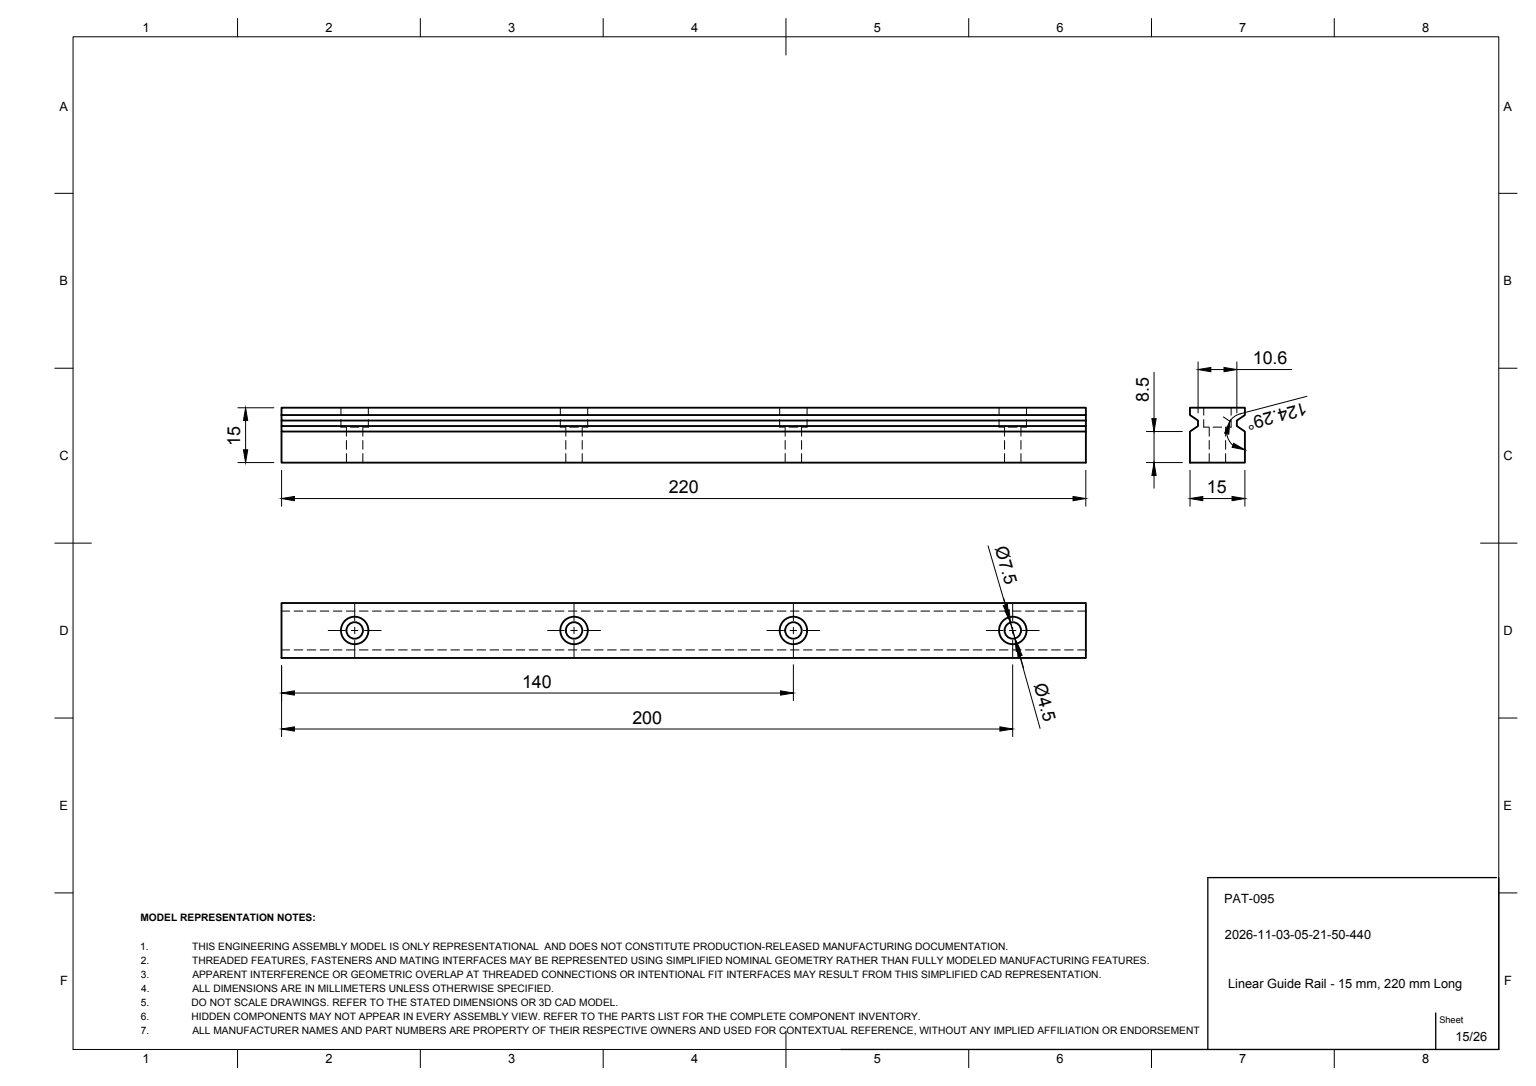
ISO-10303-21;
HEADER;
/* Generated by software containing ST-Developer
 * from STEP Tools, Inc. (www.steptools.com) 
 */

FILE_DESCRIPTION(
/* description */ ('Single-Axis Profile-Rail Linear Slide'),
/* implementation_level */ '2;1');

FILE_NAME(
/* name */ 'Linear Guide Rail - 15 mm, 220 mm Long.step',
/* time_stamp */ '2026-10-27T10:47:43-07:00',
/* author */ (''),
/* organization */ (''),
/* preprocessor_version */ 'ST-DEVELOPER v20.2',
/* originating_system */ 'Autodesk Translation Framework v15.17.0.0',
/* authorisation */ '');

FILE_SCHEMA (('AUTOMOTIVE_DESIGN { 1 0 10303 214 3 1 1 }'));
ENDSEC;

DATA;
#10=MECHANICAL_DESIGN_GEOMETRIC_PRESENTATION_REPRESENTATION('',(#339),#14478);
#285=SHAPE_REPRESENTATION_RELATIONSHIP('SRR','None',#14615,#312);
#312=ADVANCED_BREP_SHAPE_REPRESENTATION('',(#366),#14459);
#339=STYLED_ITEM('',(#14824),#366);
#366=MANIFOLD_SOLID_BREP('Body1',#8599);
#422=FACE_BOUND('',#1545,.T.);
#423=FACE_BOUND('',#1548,.T.);
#424=FACE_BOUND('',#1551,.T.);
#425=FACE_BOUND('',#1554,.T.);
#426=FACE_BOUND('',#1564,.T.);
#427=FACE_BOUND('',#1565,.T.);
#428=FACE_BOUND('',#1566,.T.);
#429=FACE_BOUND('',#1567,.T.);
#430=FACE_BOUND('',#1574,.T.);
#431=FACE_BOUND('',#1575,.T.);
#432=FACE_BOUND('',#1576,.T.);
#433=FACE_BOUND('',#1577,.T.);
#648=PLANE('',#9187);
#649=PLANE('',#9192);
#650=PLANE('',#9197);
#651=PLANE('',#9202);
#652=PLANE('',#9212);
#653=PLANE('',#9213);
#654=PLANE('',#9214);
#655=PLANE('',#9215);
#656=PLANE('',#9216);
#657=PLANE('',#9217);
#658=PLANE('',#9218);
#659=PLANE('',#9219);
#660=PLANE('',#9220);
#661=PLANE('',#9221);
#662=PLANE('',#9222);
#663=PLANE('',#9223);
#664=PLANE('',#9224);
#665=PLANE('',#9225);
#1044=FACE_OUTER_BOUND('',#1543,.T.);
#1045=FACE_OUTER_BOUND('',#1544,.T.);
#1046=FACE_OUTER_BOUND('',#1546,.T.);
#1047=FACE_OUTER_BOUND('',#1547,.T.);
#1048=FACE_OUTER_BOUND('',#1549,.T.);
#1049=FACE_OUTER_BOUND('',#1550,.T.);
#1050=FACE_OUTER_BOUND('',#1552,.T.);
#1051=FACE_OUTER_BOUND('',#1553,.T.);
#1052=FACE_OUTER_BOUND('',#1555,.T.);
#1053=FACE_OUTER_BOUND('',#1556,.T.);
#1054=FACE_OUTER_BOUND('',#1557,.T.);
#1055=FACE_OUTER_BOUND('',#1558,.T.);
#1056=FACE_OUTER_BOUND('',#1559,.T.);
#1057=FACE_OUTER_BOUND('',#1560,.T.);
#1058=FACE_OUTER_BOUND('',#1561,.T.);
#1059=FACE_OUTER_BOUND('',#1562,.T.);
#1060=FACE_OUTER_BOUND('',#1563,.T.);
#1061=FACE_OUTER_BOUND('',#1568,.T.);
#1062=FACE_OUTER_BOUND('',#1569,.T.);
#1063=FACE_OUTER_BOUND('',#1570,.T.);
#1064=FACE_OUTER_BOUND('',#1571,.T.);
#1065=FACE_OUTER_BOUND('',#1572,.T.);
#1066=FACE_OUTER_BOUND('',#1573,.T.);
#1067=FACE_OUTER_BOUND('',#1578,.T.);
#1068=FACE_OUTER_BOUND('',#1579,.T.);
#1069=FACE_OUTER_BOUND('',#1580,.T.);
#1543=EDGE_LOOP('',(#6893,#6894,#6895,#6896));
#1544=EDGE_LOOP('',(#6897));
#1545=EDGE_LOOP('',(#6898));
#1546=EDGE_LOOP('',(#6899,#6900,#6901,#6902));
#1547=EDGE_LOOP('',(#6903));
#1548=EDGE_LOOP('',(#6904));
#1549=EDGE_LOOP('',(#6905,#6906,#6907,#6908));
#1550=EDGE_LOOP('',(#6909));
#1551=EDGE_LOOP('',(#6910));
#1552=EDGE_LOOP('',(#6911,#6912,#6913,#6914));
#1553=EDGE_LOOP('',(#6915));
#1554=EDGE_LOOP('',(#6916));
#1555=EDGE_LOOP('',(#6917,#6918,#6919,#6920));
#1556=EDGE_LOOP('',(#6921,#6922,#6923,#6924));
#1557=EDGE_LOOP('',(#6925,#6926,#6927,#6928));
#1558=EDGE_LOOP('',(#6929,#6930,#6931,#6932));
#1559=EDGE_LOOP('',(#6933,#6934,#6935,#6936));
#1560=EDGE_LOOP('',(#6937,#6938,#6939,#6940));
#1561=EDGE_LOOP('',(#6941,#6942,#6943,#6944));
#1562=EDGE_LOOP('',(#6945,#6946,#6947,#6948));
#1563=EDGE_LOOP('',(#6949,#6950,#6951,#6952));
#1564=EDGE_LOOP('',(#6953));
#1565=EDGE_LOOP('',(#6954));
#1566=EDGE_LOOP('',(#6955));
#1567=EDGE_LOOP('',(#6956));
#1568=EDGE_LOOP('',(#6957,#6958,#6959,#6960));
#1569=EDGE_LOOP('',(#6961,#6962,#6963,#6964));
#1570=EDGE_LOOP('',(#6965,#6966,#6967,#6968));
#1571=EDGE_LOOP('',(#6969,#6970,#6971,#6972));
#1572=EDGE_LOOP('',(#6973,#6974,#6975,#6976));
#1573=EDGE_LOOP('',(#6977,#6978,#6979,#6980));
#1574=EDGE_LOOP('',(#6981));
#1575=EDGE_LOOP('',(#6982));
#1576=EDGE_LOOP('',(#6983));
#1577=EDGE_LOOP('',(#6984));
#1578=EDGE_LOOP('',(#6985,#6986,#6987,#6988));
#1579=EDGE_LOOP('',(#6989,#6990,#6991,#6992,#6993,#6994,#6995,#6996,#6997,
#6998,#6999,#7000));
#1580=EDGE_LOOP('',(#7001,#7002,#7003,#7004,#7005,#7006,#7007,#7008,#7009,
#7010,#7011,#7012));
#2332=LINE('',#13117,#3303);
#2333=LINE('',#13126,#3304);
#2334=LINE('',#13135,#3305);
#2335=LINE('',#13144,#3306);
#2336=LINE('',#13152,#3307);
#2337=LINE('',#13156,#3308);
#2338=LINE('',#13160,#3309);
#2339=LINE('',#13164,#3310);
#2340=LINE('',#13168,#3311);
#2341=LINE('',#13170,#3312);
#2342=LINE('',#13172,#3313);
#2343=LINE('',#13173,#3314);
#2344=LINE('',#13176,#3315);
#2345=LINE('',#13178,#3316);
#2346=LINE('',#13179,#3317);
#2347=LINE('',#13182,#3318);
#2348=LINE('',#13184,#3319);
#2349=LINE('',#13185,#3320);
#2350=LINE('',#13188,#3321);
#2351=LINE('',#13190,#3322);
#2352=LINE('',#13191,#3323);
#2353=LINE('',#13194,#3324);
#2354=LINE('',#13196,#3325);
#2355=LINE('',#13197,#3326);
#2356=LINE('',#13200,#3327);
#2357=LINE('',#13202,#3328);
#2358=LINE('',#13203,#3329);
#2359=LINE('',#13206,#3330);
#2360=LINE('',#13208,#3331);
#2361=LINE('',#13209,#3332);
#2362=LINE('',#13212,#3333);
#2363=LINE('',#13214,#3334);
#2364=LINE('',#13215,#3335);
#2365=LINE('',#13218,#3336);
#2366=LINE('',#13220,#3337);
#2367=LINE('',#13221,#3338);
#2368=LINE('',#13224,#3339);
#2369=LINE('',#13226,#3340);
#2370=LINE('',#13227,#3341);
#2371=LINE('',#13230,#3342);
#2372=LINE('',#13232,#3343);
#2373=LINE('',#13233,#3344);
#2374=LINE('',#13235,#3345);
#2375=LINE('',#13236,#3346);
#3303=VECTOR('',#10647,0.375);
#3304=VECTOR('',#10658,0.375);
#3305=VECTOR('',#10669,0.375);
#3306=VECTOR('',#10680,0.375);
#3307=VECTOR('',#10691,0.225);
#3308=VECTOR('',#10696,0.225);
#3309=VECTOR('',#10701,0.225);
#3310=VECTOR('',#10706,0.225000000000001);
#3311=VECTOR('',#10709,1.);
#3312=VECTOR('',#10710,1.);
#3313=VECTOR('',#10711,1.);
#3314=VECTOR('',#10712,1.);
#3315=VECTOR('',#10715,1.);
#3316=VECTOR('',#10716,1.);
#3317=VECTOR('',#10717,1.);
#3318=VECTOR('',#10720,1.);
#3319=VECTOR('',#10721,1.);
#3320=VECTOR('',#10722,1.);
#3321=VECTOR('',#10725,1.);
#3322=VECTOR('',#10726,1.);
#3323=VECTOR('',#10727,1.);
#3324=VECTOR('',#10730,1.);
#3325=VECTOR('',#10731,1.);
#3326=VECTOR('',#10732,1.);
#3327=VECTOR('',#10735,1.);
#3328=VECTOR('',#10736,1.);
#3329=VECTOR('',#10737,1.);
#3330=VECTOR('',#10740,1.);
#3331=VECTOR('',#10741,1.);
#3332=VECTOR('',#10742,1.);
#3333=VECTOR('',#10745,1.);
#3334=VECTOR('',#10746,1.);
#3335=VECTOR('',#10747,1.);
#3336=VECTOR('',#10750,1.);
#3337=VECTOR('',#10751,1.);
#3338=VECTOR('',#10752,1.);
#3339=VECTOR('',#10755,1.);
#3340=VECTOR('',#10756,1.);
#3341=VECTOR('',#10757,1.);
#3342=VECTOR('',#10760,1.);
#3343=VECTOR('',#10761,1.);
#3344=VECTOR('',#10762,1.);
#3345=VECTOR('',#10765,1.);
#3346=VECTOR('',#10766,1.);
#3830=CIRCLE('',#9185,0.375);
#3831=CIRCLE('',#9186,0.375);
#3832=CIRCLE('',#9188,0.225);
#3833=CIRCLE('',#9190,0.375);
#3834=CIRCLE('',#9191,0.375);
#3835=CIRCLE('',#9193,0.225);
#3836=CIRCLE('',#9195,0.375);
#3837=CIRCLE('',#9196,0.375);
#3838=CIRCLE('',#9198,0.225);
#3839=CIRCLE('',#9200,0.375);
#3840=CIRCLE('',#9201,0.375);
#3841=CIRCLE('',#9203,0.225000000000001);
#3842=CIRCLE('',#9205,0.225);
#3843=CIRCLE('',#9207,0.225);
#3844=CIRCLE('',#9209,0.225);
#3845=CIRCLE('',#9211,0.225000000000001);
#4298=VERTEX_POINT('',#13114);
#4299=VERTEX_POINT('',#13116);
#4300=VERTEX_POINT('',#13120);
#4301=VERTEX_POINT('',#13123);
#4302=VERTEX_POINT('',#13125);
#4303=VERTEX_POINT('',#13129);
#4304=VERTEX_POINT('',#13132);
#4305=VERTEX_POINT('',#13134);
#4306=VERTEX_POINT('',#13138);
#4307=VERTEX_POINT('',#13141);
#4308=VERTEX_POINT('',#13143);
#4309=VERTEX_POINT('',#13147);
#4310=VERTEX_POINT('',#13150);
#4311=VERTEX_POINT('',#13154);
#4312=VERTEX_POINT('',#13158);
#4313=VERTEX_POINT('',#13162);
#4314=VERTEX_POINT('',#13166);
#4315=VERTEX_POINT('',#13167);
#4316=VERTEX_POINT('',#13169);
#4317=VERTEX_POINT('',#13171);
#4318=VERTEX_POINT('',#13175);
#4319=VERTEX_POINT('',#13177);
#4320=VERTEX_POINT('',#13181);
#4321=VERTEX_POINT('',#13183);
#4322=VERTEX_POINT('',#13187);
#4323=VERTEX_POINT('',#13189);
#4324=VERTEX_POINT('',#13193);
#4325=VERTEX_POINT('',#13195);
#4326=VERTEX_POINT('',#13199);
#4327=VERTEX_POINT('',#13201);
#4328=VERTEX_POINT('',#13205);
#4329=VERTEX_POINT('',#13207);
#4330=VERTEX_POINT('',#13211);
#4331=VERTEX_POINT('',#13213);
#4332=VERTEX_POINT('',#13217);
#4333=VERTEX_POINT('',#13219);
#4334=VERTEX_POINT('',#13223);
#4335=VERTEX_POINT('',#13225);
#4336=VERTEX_POINT('',#13229);
#4337=VERTEX_POINT('',#13231);
#5224=EDGE_CURVE('',#4298,#4298,#3830,.T.);
#5225=EDGE_CURVE('',#4298,#4299,#2332,.T.);
#5226=EDGE_CURVE('',#4299,#4299,#3831,.T.);
#5227=EDGE_CURVE('',#4300,#4300,#3832,.T.);
#5228=EDGE_CURVE('',#4301,#4301,#3833,.T.);
#5229=EDGE_CURVE('',#4301,#4302,#2333,.T.);
#5230=EDGE_CURVE('',#4302,#4302,#3834,.T.);
#5231=EDGE_CURVE('',#4303,#4303,#3835,.T.);
#5232=EDGE_CURVE('',#4304,#4304,#3836,.T.);
#5233=EDGE_CURVE('',#4304,#4305,#2334,.T.);
#5234=EDGE_CURVE('',#4305,#4305,#3837,.T.);
#5235=EDGE_CURVE('',#4306,#4306,#3838,.T.);
#5236=EDGE_CURVE('',#4307,#4307,#3839,.T.);
#5237=EDGE_CURVE('',#4307,#4308,#2335,.T.);
#5238=EDGE_CURVE('',#4308,#4308,#3840,.T.);
#5239=EDGE_CURVE('',#4309,#4309,#3841,.T.);
#5240=EDGE_CURVE('',#4310,#4310,#3842,.T.);
#5241=EDGE_CURVE('',#4310,#4300,#2336,.T.);
#5242=EDGE_CURVE('',#4311,#4311,#3843,.T.);
#5243=EDGE_CURVE('',#4311,#4303,#2337,.T.);
#5244=EDGE_CURVE('',#4312,#4312,#3844,.T.);
#5245=EDGE_CURVE('',#4312,#4306,#2338,.T.);
#5246=EDGE_CURVE('',#4313,#4313,#3845,.T.);
#5247=EDGE_CURVE('',#4313,#4309,#2339,.T.);
#5248=EDGE_CURVE('',#4314,#4315,#2340,.T.);
#5249=EDGE_CURVE('',#4315,#4316,#2341,.T.);
#5250=EDGE_CURVE('',#4317,#4316,#2342,.T.);
#5251=EDGE_CURVE('',#4314,#4317,#2343,.T.);
#5252=EDGE_CURVE('',#4318,#4314,#2344,.T.);
#5253=EDGE_CURVE('',#4319,#4317,#2345,.T.);
#5254=EDGE_CURVE('',#4318,#4319,#2346,.T.);
#5255=EDGE_CURVE('',#4320,#4318,#2347,.T.);
#5256=EDGE_CURVE('',#4321,#4319,#2348,.T.);
#5257=EDGE_CURVE('',#4320,#4321,#2349,.T.);
#5258=EDGE_CURVE('',#4322,#4320,#2350,.T.);
#5259=EDGE_CURVE('',#4323,#4321,#2351,.T.);
#5260=EDGE_CURVE('',#4322,#4323,#2352,.T.);
#5261=EDGE_CURVE('',#4324,#4322,#2353,.T.);
#5262=EDGE_CURVE('',#4325,#4323,#2354,.T.);
#5263=EDGE_CURVE('',#4324,#4325,#2355,.T.);
#5264=EDGE_CURVE('',#4326,#4324,#2356,.T.);
#5265=EDGE_CURVE('',#4327,#4325,#2357,.T.);
#5266=EDGE_CURVE('',#4326,#4327,#2358,.T.);
#5267=EDGE_CURVE('',#4328,#4326,#2359,.T.);
#5268=EDGE_CURVE('',#4329,#4327,#2360,.T.);
#5269=EDGE_CURVE('',#4328,#4329,#2361,.T.);
#5270=EDGE_CURVE('',#4330,#4328,#2362,.T.);
#5271=EDGE_CURVE('',#4331,#4329,#2363,.T.);
#5272=EDGE_CURVE('',#4330,#4331,#2364,.T.);
#5273=EDGE_CURVE('',#4332,#4330,#2365,.T.);
#5274=EDGE_CURVE('',#4333,#4331,#2366,.T.);
#5275=EDGE_CURVE('',#4332,#4333,#2367,.T.);
#5276=EDGE_CURVE('',#4334,#4332,#2368,.T.);
#5277=EDGE_CURVE('',#4335,#4333,#2369,.T.);
#5278=EDGE_CURVE('',#4334,#4335,#2370,.T.);
#5279=EDGE_CURVE('',#4336,#4334,#2371,.T.);
#5280=EDGE_CURVE('',#4337,#4335,#2372,.T.);
#5281=EDGE_CURVE('',#4336,#4337,#2373,.T.);
#5282=EDGE_CURVE('',#4315,#4336,#2374,.T.);
#5283=EDGE_CURVE('',#4316,#4337,#2375,.T.);
#6893=ORIENTED_EDGE('',*,*,#5224,.F.);
#6894=ORIENTED_EDGE('',*,*,#5225,.T.);
#6895=ORIENTED_EDGE('',*,*,#5226,.F.);
#6896=ORIENTED_EDGE('',*,*,#5225,.F.);
#6897=ORIENTED_EDGE('',*,*,#5224,.T.);
#6898=ORIENTED_EDGE('',*,*,#5227,.F.);
#6899=ORIENTED_EDGE('',*,*,#5228,.F.);
#6900=ORIENTED_EDGE('',*,*,#5229,.T.);
#6901=ORIENTED_EDGE('',*,*,#5230,.F.);
#6902=ORIENTED_EDGE('',*,*,#5229,.F.);
#6903=ORIENTED_EDGE('',*,*,#5228,.T.);
#6904=ORIENTED_EDGE('',*,*,#5231,.F.);
#6905=ORIENTED_EDGE('',*,*,#5232,.F.);
#6906=ORIENTED_EDGE('',*,*,#5233,.T.);
#6907=ORIENTED_EDGE('',*,*,#5234,.F.);
#6908=ORIENTED_EDGE('',*,*,#5233,.F.);
#6909=ORIENTED_EDGE('',*,*,#5232,.T.);
#6910=ORIENTED_EDGE('',*,*,#5235,.F.);
#6911=ORIENTED_EDGE('',*,*,#5236,.F.);
#6912=ORIENTED_EDGE('',*,*,#5237,.T.);
#6913=ORIENTED_EDGE('',*,*,#5238,.F.);
#6914=ORIENTED_EDGE('',*,*,#5237,.F.);
#6915=ORIENTED_EDGE('',*,*,#5236,.T.);
#6916=ORIENTED_EDGE('',*,*,#5239,.F.);
#6917=ORIENTED_EDGE('',*,*,#5240,.F.);
#6918=ORIENTED_EDGE('',*,*,#5241,.T.);
#6919=ORIENTED_EDGE('',*,*,#5227,.T.);
#6920=ORIENTED_EDGE('',*,*,#5241,.F.);
#6921=ORIENTED_EDGE('',*,*,#5242,.F.);
#6922=ORIENTED_EDGE('',*,*,#5243,.T.);
#6923=ORIENTED_EDGE('',*,*,#5231,.T.);
#6924=ORIENTED_EDGE('',*,*,#5243,.F.);
#6925=ORIENTED_EDGE('',*,*,#5244,.F.);
#6926=ORIENTED_EDGE('',*,*,#5245,.T.);
#6927=ORIENTED_EDGE('',*,*,#5235,.T.);
#6928=ORIENTED_EDGE('',*,*,#5245,.F.);
#6929=ORIENTED_EDGE('',*,*,#5246,.F.);
#6930=ORIENTED_EDGE('',*,*,#5247,.T.);
#6931=ORIENTED_EDGE('',*,*,#5239,.T.);
#6932=ORIENTED_EDGE('',*,*,#5247,.F.);
#6933=ORIENTED_EDGE('',*,*,#5248,.T.);
#6934=ORIENTED_EDGE('',*,*,#5249,.T.);
#6935=ORIENTED_EDGE('',*,*,#5250,.F.);
#6936=ORIENTED_EDGE('',*,*,#5251,.F.);
#6937=ORIENTED_EDGE('',*,*,#5252,.T.);
#6938=ORIENTED_EDGE('',*,*,#5251,.T.);
#6939=ORIENTED_EDGE('',*,*,#5253,.F.);
#6940=ORIENTED_EDGE('',*,*,#5254,.F.);
#6941=ORIENTED_EDGE('',*,*,#5255,.T.);
#6942=ORIENTED_EDGE('',*,*,#5254,.T.);
#6943=ORIENTED_EDGE('',*,*,#5256,.F.);
#6944=ORIENTED_EDGE('',*,*,#5257,.F.);
#6945=ORIENTED_EDGE('',*,*,#5258,.T.);
#6946=ORIENTED_EDGE('',*,*,#5257,.T.);
#6947=ORIENTED_EDGE('',*,*,#5259,.F.);
#6948=ORIENTED_EDGE('',*,*,#5260,.F.);
#6949=ORIENTED_EDGE('',*,*,#5261,.T.);
#6950=ORIENTED_EDGE('',*,*,#5260,.T.);
#6951=ORIENTED_EDGE('',*,*,#5262,.F.);
#6952=ORIENTED_EDGE('',*,*,#5263,.F.);
#6953=ORIENTED_EDGE('',*,*,#5238,.T.);
#6954=ORIENTED_EDGE('',*,*,#5234,.T.);
#6955=ORIENTED_EDGE('',*,*,#5230,.T.);
#6956=ORIENTED_EDGE('',*,*,#5226,.T.);
#6957=ORIENTED_EDGE('',*,*,#5264,.T.);
#6958=ORIENTED_EDGE('',*,*,#5263,.T.);
#6959=ORIENTED_EDGE('',*,*,#5265,.F.);
#6960=ORIENTED_EDGE('',*,*,#5266,.F.);
#6961=ORIENTED_EDGE('',*,*,#5267,.T.);
#6962=ORIENTED_EDGE('',*,*,#5266,.T.);
#6963=ORIENTED_EDGE('',*,*,#5268,.F.);
#6964=ORIENTED_EDGE('',*,*,#5269,.F.);
#6965=ORIENTED_EDGE('',*,*,#5270,.T.);
#6966=ORIENTED_EDGE('',*,*,#5269,.T.);
#6967=ORIENTED_EDGE('',*,*,#5271,.F.);
#6968=ORIENTED_EDGE('',*,*,#5272,.F.);
#6969=ORIENTED_EDGE('',*,*,#5273,.T.);
#6970=ORIENTED_EDGE('',*,*,#5272,.T.);
#6971=ORIENTED_EDGE('',*,*,#5274,.F.);
#6972=ORIENTED_EDGE('',*,*,#5275,.F.);
#6973=ORIENTED_EDGE('',*,*,#5276,.T.);
#6974=ORIENTED_EDGE('',*,*,#5275,.T.);
#6975=ORIENTED_EDGE('',*,*,#5277,.F.);
#6976=ORIENTED_EDGE('',*,*,#5278,.F.);
#6977=ORIENTED_EDGE('',*,*,#5279,.T.);
#6978=ORIENTED_EDGE('',*,*,#5278,.T.);
#6979=ORIENTED_EDGE('',*,*,#5280,.F.);
#6980=ORIENTED_EDGE('',*,*,#5281,.F.);
#6981=ORIENTED_EDGE('',*,*,#5240,.T.);
#6982=ORIENTED_EDGE('',*,*,#5242,.T.);
#6983=ORIENTED_EDGE('',*,*,#5244,.T.);
#6984=ORIENTED_EDGE('',*,*,#5246,.T.);
#6985=ORIENTED_EDGE('',*,*,#5282,.T.);
#6986=ORIENTED_EDGE('',*,*,#5281,.T.);
#6987=ORIENTED_EDGE('',*,*,#5283,.F.);
#6988=ORIENTED_EDGE('',*,*,#5249,.F.);
#6989=ORIENTED_EDGE('',*,*,#5283,.T.);
#6990=ORIENTED_EDGE('',*,*,#5280,.T.);
#6991=ORIENTED_EDGE('',*,*,#5277,.T.);
#6992=ORIENTED_EDGE('',*,*,#5274,.T.);
#6993=ORIENTED_EDGE('',*,*,#5271,.T.);
#6994=ORIENTED_EDGE('',*,*,#5268,.T.);
#6995=ORIENTED_EDGE('',*,*,#5265,.T.);
#6996=ORIENTED_EDGE('',*,*,#5262,.T.);
#6997=ORIENTED_EDGE('',*,*,#5259,.T.);
#6998=ORIENTED_EDGE('',*,*,#5256,.T.);
#6999=ORIENTED_EDGE('',*,*,#5253,.T.);
#7000=ORIENTED_EDGE('',*,*,#5250,.T.);
#7001=ORIENTED_EDGE('',*,*,#5282,.F.);
#7002=ORIENTED_EDGE('',*,*,#5248,.F.);
#7003=ORIENTED_EDGE('',*,*,#5252,.F.);
#7004=ORIENTED_EDGE('',*,*,#5255,.F.);
#7005=ORIENTED_EDGE('',*,*,#5258,.F.);
#7006=ORIENTED_EDGE('',*,*,#5261,.F.);
#7007=ORIENTED_EDGE('',*,*,#5264,.F.);
#7008=ORIENTED_EDGE('',*,*,#5267,.F.);
#7009=ORIENTED_EDGE('',*,*,#5270,.F.);
#7010=ORIENTED_EDGE('',*,*,#5273,.F.);
#7011=ORIENTED_EDGE('',*,*,#5276,.F.);
#7012=ORIENTED_EDGE('',*,*,#5279,.F.);
#8095=CYLINDRICAL_SURFACE('',#9184,0.375);
#8096=CYLINDRICAL_SURFACE('',#9189,0.375);
#8097=CYLINDRICAL_SURFACE('',#9194,0.375);
#8098=CYLINDRICAL_SURFACE('',#9199,0.375);
#8099=CYLINDRICAL_SURFACE('',#9204,0.225);
#8100=CYLINDRICAL_SURFACE('',#9206,0.225);
#8101=CYLINDRICAL_SURFACE('',#9208,0.225);
#8102=CYLINDRICAL_SURFACE('',#9210,0.225000000000001);
#8338=ADVANCED_FACE('',(#1044),#8095,.F.);
#8339=ADVANCED_FACE('',(#1045,#422),#648,.T.);
#8340=ADVANCED_FACE('',(#1046),#8096,.F.);
#8341=ADVANCED_FACE('',(#1047,#423),#649,.T.);
#8342=ADVANCED_FACE('',(#1048),#8097,.F.);
#8343=ADVANCED_FACE('',(#1049,#424),#650,.T.);
#8344=ADVANCED_FACE('',(#1050),#8098,.F.);
#8345=ADVANCED_FACE('',(#1051,#425),#651,.T.);
#8346=ADVANCED_FACE('',(#1052),#8099,.F.);
#8347=ADVANCED_FACE('',(#1053),#8100,.F.);
#8348=ADVANCED_FACE('',(#1054),#8101,.F.);
#8349=ADVANCED_FACE('',(#1055),#8102,.F.);
#8350=ADVANCED_FACE('',(#1056),#652,.T.);
#8351=ADVANCED_FACE('',(#1057),#653,.T.);
#8352=ADVANCED_FACE('',(#1058),#654,.T.);
#8353=ADVANCED_FACE('',(#1059),#655,.T.);
#8354=ADVANCED_FACE('',(#1060,#426,#427,#428,#429),#656,.T.);
#8355=ADVANCED_FACE('',(#1061),#657,.T.);
#8356=ADVANCED_FACE('',(#1062),#658,.T.);
#8357=ADVANCED_FACE('',(#1063),#659,.T.);
#8358=ADVANCED_FACE('',(#1064),#660,.T.);
#8359=ADVANCED_FACE('',(#1065),#661,.T.);
#8360=ADVANCED_FACE('',(#1066,#430,#431,#432,#433),#662,.T.);
#8361=ADVANCED_FACE('',(#1067),#663,.T.);
#8362=ADVANCED_FACE('',(#1068),#664,.T.);
#8363=ADVANCED_FACE('',(#1069),#665,.F.);
#8599=CLOSED_SHELL('',(#8338,#8339,#8340,#8341,#8342,#8343,#8344,#8345,
#8346,#8347,#8348,#8349,#8350,#8351,#8352,#8353,#8354,#8355,#8356,#8357,
#8358,#8359,#8360,#8361,#8362,#8363));
#9183=AXIS2_PLACEMENT_3D('',#13112,#10641,#10642);
#9184=AXIS2_PLACEMENT_3D('',#13113,#10643,#10644);
#9185=AXIS2_PLACEMENT_3D('',#13115,#10645,#10646);
#9186=AXIS2_PLACEMENT_3D('',#13118,#10648,#10649);
#9187=AXIS2_PLACEMENT_3D('',#13119,#10650,#10651);
#9188=AXIS2_PLACEMENT_3D('',#13121,#10652,#10653);
#9189=AXIS2_PLACEMENT_3D('',#13122,#10654,#10655);
#9190=AXIS2_PLACEMENT_3D('',#13124,#10656,#10657);
#9191=AXIS2_PLACEMENT_3D('',#13127,#10659,#10660);
#9192=AXIS2_PLACEMENT_3D('',#13128,#10661,#10662);
#9193=AXIS2_PLACEMENT_3D('',#13130,#10663,#10664);
#9194=AXIS2_PLACEMENT_3D('',#13131,#10665,#10666);
#9195=AXIS2_PLACEMENT_3D('',#13133,#10667,#10668);
#9196=AXIS2_PLACEMENT_3D('',#13136,#10670,#10671);
#9197=AXIS2_PLACEMENT_3D('',#13137,#10672,#10673);
#9198=AXIS2_PLACEMENT_3D('',#13139,#10674,#10675);
#9199=AXIS2_PLACEMENT_3D('',#13140,#10676,#10677);
#9200=AXIS2_PLACEMENT_3D('',#13142,#10678,#10679);
#9201=AXIS2_PLACEMENT_3D('',#13145,#10681,#10682);
#9202=AXIS2_PLACEMENT_3D('',#13146,#10683,#10684);
#9203=AXIS2_PLACEMENT_3D('',#13148,#10685,#10686);
#9204=AXIS2_PLACEMENT_3D('',#13149,#10687,#10688);
#9205=AXIS2_PLACEMENT_3D('',#13151,#10689,#10690);
#9206=AXIS2_PLACEMENT_3D('',#13153,#10692,#10693);
#9207=AXIS2_PLACEMENT_3D('',#13155,#10694,#10695);
#9208=AXIS2_PLACEMENT_3D('',#13157,#10697,#10698);
#9209=AXIS2_PLACEMENT_3D('',#13159,#10699,#10700);
#9210=AXIS2_PLACEMENT_3D('',#13161,#10702,#10703);
#9211=AXIS2_PLACEMENT_3D('',#13163,#10704,#10705);
#9212=AXIS2_PLACEMENT_3D('',#13165,#10707,#10708);
#9213=AXIS2_PLACEMENT_3D('',#13174,#10713,#10714);
#9214=AXIS2_PLACEMENT_3D('',#13180,#10718,#10719);
#9215=AXIS2_PLACEMENT_3D('',#13186,#10723,#10724);
#9216=AXIS2_PLACEMENT_3D('',#13192,#10728,#10729);
#9217=AXIS2_PLACEMENT_3D('',#13198,#10733,#10734);
#9218=AXIS2_PLACEMENT_3D('',#13204,#10738,#10739);
#9219=AXIS2_PLACEMENT_3D('',#13210,#10743,#10744);
#9220=AXIS2_PLACEMENT_3D('',#13216,#10748,#10749);
#9221=AXIS2_PLACEMENT_3D('',#13222,#10753,#10754);
#9222=AXIS2_PLACEMENT_3D('',#13228,#10758,#10759);
#9223=AXIS2_PLACEMENT_3D('',#13234,#10763,#10764);
#9224=AXIS2_PLACEMENT_3D('',#13237,#10767,#10768);
#9225=AXIS2_PLACEMENT_3D('',#13238,#10769,#10770);
#10641=DIRECTION('axis',(0.,0.,1.));
#10642=DIRECTION('refdir',(1.,0.,0.));
#10643=DIRECTION('center_axis',(0.,0.,1.));
#10644=DIRECTION('ref_axis',(1.,0.,0.));
#10645=DIRECTION('center_axis',(0.,0.,1.));
#10646=DIRECTION('ref_axis',(1.,0.,0.));
#10647=DIRECTION('',(0.,0.,1.));
#10648=DIRECTION('center_axis',(0.,0.,-1.));
#10649=DIRECTION('ref_axis',(1.,0.,0.));
#10650=DIRECTION('center_axis',(0.,0.,1.));
#10651=DIRECTION('ref_axis',(1.,0.,0.));
#10652=DIRECTION('center_axis',(0.,0.,1.));
#10653=DIRECTION('ref_axis',(1.,0.,0.));
#10654=DIRECTION('center_axis',(0.,0.,1.));
#10655=DIRECTION('ref_axis',(1.,0.,0.));
#10656=DIRECTION('center_axis',(0.,0.,1.));
#10657=DIRECTION('ref_axis',(1.,0.,0.));
#10658=DIRECTION('',(0.,0.,1.));
#10659=DIRECTION('center_axis',(0.,0.,-1.));
#10660=DIRECTION('ref_axis',(1.,0.,0.));
#10661=DIRECTION('center_axis',(0.,0.,1.));
#10662=DIRECTION('ref_axis',(1.,0.,0.));
#10663=DIRECTION('center_axis',(0.,0.,1.));
#10664=DIRECTION('ref_axis',(1.,0.,0.));
#10665=DIRECTION('center_axis',(0.,0.,1.));
#10666=DIRECTION('ref_axis',(1.,0.,0.));
#10667=DIRECTION('center_axis',(0.,0.,1.));
#10668=DIRECTION('ref_axis',(1.,0.,0.));
#10669=DIRECTION('',(0.,0.,1.));
#10670=DIRECTION('center_axis',(0.,0.,-1.));
#10671=DIRECTION('ref_axis',(1.,0.,0.));
#10672=DIRECTION('center_axis',(0.,0.,1.));
#10673=DIRECTION('ref_axis',(1.,0.,0.));
#10674=DIRECTION('center_axis',(0.,0.,1.));
#10675=DIRECTION('ref_axis',(1.,0.,0.));
#10676=DIRECTION('center_axis',(0.,0.,1.));
#10677=DIRECTION('ref_axis',(1.,0.,0.));
#10678=DIRECTION('center_axis',(0.,0.,1.));
#10679=DIRECTION('ref_axis',(1.,0.,0.));
#10680=DIRECTION('',(0.,0.,1.));
#10681=DIRECTION('center_axis',(0.,0.,-1.));
#10682=DIRECTION('ref_axis',(1.,0.,0.));
#10683=DIRECTION('center_axis',(0.,0.,1.));
#10684=DIRECTION('ref_axis',(1.,0.,0.));
#10685=DIRECTION('center_axis',(0.,0.,1.));
#10686=DIRECTION('ref_axis',(1.,0.,0.));
#10687=DIRECTION('center_axis',(0.,0.,1.));
#10688=DIRECTION('ref_axis',(1.,0.,0.));
#10689=DIRECTION('center_axis',(0.,0.,1.));
#10690=DIRECTION('ref_axis',(1.,0.,0.));
#10691=DIRECTION('',(0.,0.,1.));
#10692=DIRECTION('center_axis',(0.,0.,1.));
#10693=DIRECTION('ref_axis',(1.,0.,0.));
#10694=DIRECTION('center_axis',(0.,0.,1.));
#10695=DIRECTION('ref_axis',(1.,0.,0.));
#10696=DIRECTION('',(0.,0.,1.));
#10697=DIRECTION('center_axis',(0.,0.,1.));
#10698=DIRECTION('ref_axis',(1.,0.,0.));
#10699=DIRECTION('center_axis',(0.,0.,1.));
#10700=DIRECTION('ref_axis',(1.,0.,0.));
#10701=DIRECTION('',(0.,0.,1.));
#10702=DIRECTION('center_axis',(0.,0.,1.));
#10703=DIRECTION('ref_axis',(1.,0.,0.));
#10704=DIRECTION('center_axis',(0.,0.,1.));
#10705=DIRECTION('ref_axis',(1.,0.,0.));
#10706=DIRECTION('',(0.,0.,1.));
#10707=DIRECTION('center_axis',(0.,-0.56333682464151,0.826227342807548));
#10708=DIRECTION('ref_axis',(0.,-0.826227342807548,-0.56333682464151));
#10709=DIRECTION('',(0.,-0.826227342807548,-0.56333682464151));
#10710=DIRECTION('',(1.,0.,0.));
#10711=DIRECTION('',(0.,-0.826227342807548,-0.56333682464151));
#10712=DIRECTION('',(1.,0.,0.));
#10713=DIRECTION('center_axis',(0.,-1.,0.));
#10714=DIRECTION('ref_axis',(0.,0.,-1.));
#10715=DIRECTION('',(0.,0.,-1.));
#10716=DIRECTION('',(0.,0.,-1.));
#10717=DIRECTION('',(1.,0.,0.));
#10718=DIRECTION('center_axis',(0.,-0.56333682464151,-0.826227342807548));
#10719=DIRECTION('ref_axis',(0.,0.826227342807548,-0.56333682464151));
#10720=DIRECTION('',(0.,0.826227342807548,-0.56333682464151));
#10721=DIRECTION('',(0.,0.826227342807548,-0.56333682464151));
#10722=DIRECTION('',(1.,0.,0.));
#10723=DIRECTION('center_axis',(0.,-1.,0.));
#10724=DIRECTION('ref_axis',(0.,0.,-1.));
#10725=DIRECTION('',(0.,0.,-1.));
#10726=DIRECTION('',(0.,0.,-1.));
#10727=DIRECTION('',(1.,0.,0.));
#10728=DIRECTION('center_axis',(0.,0.,1.));
#10729=DIRECTION('ref_axis',(0.,-1.,0.));
#10730=DIRECTION('',(0.,-1.,0.));
#10731=DIRECTION('',(0.,-1.,0.));
#10732=DIRECTION('',(1.,0.,0.));
#10733=DIRECTION('center_axis',(0.,1.,0.));
#10734=DIRECTION('ref_axis',(0.,0.,1.));
#10735=DIRECTION('',(0.,0.,1.));
#10736=DIRECTION('',(0.,0.,1.));
#10737=DIRECTION('',(1.,0.,0.));
#10738=DIRECTION('center_axis',(0.,0.56333682464151,-0.826227342807548));
#10739=DIRECTION('ref_axis',(0.,0.826227342807548,0.56333682464151));
#10740=DIRECTION('',(0.,0.826227342807548,0.56333682464151));
#10741=DIRECTION('',(0.,0.826227342807548,0.56333682464151));
#10742=DIRECTION('',(1.,0.,0.));
#10743=DIRECTION('center_axis',(0.,1.,0.));
#10744=DIRECTION('ref_axis',(0.,0.,1.));
#10745=DIRECTION('',(0.,0.,1.));
#10746=DIRECTION('',(0.,0.,1.));
#10747=DIRECTION('',(1.,0.,0.));
#10748=DIRECTION('center_axis',(0.,0.56333682464151,0.826227342807548));
#10749=DIRECTION('ref_axis',(0.,-0.826227342807548,0.56333682464151));
#10750=DIRECTION('',(0.,-0.826227342807548,0.56333682464151));
#10751=DIRECTION('',(0.,-0.826227342807548,0.56333682464151));
#10752=DIRECTION('',(1.,0.,0.));
#10753=DIRECTION('center_axis',(0.,1.,0.));
#10754=DIRECTION('ref_axis',(0.,0.,1.));
#10755=DIRECTION('',(0.,0.,1.));
#10756=DIRECTION('',(0.,0.,1.));
#10757=DIRECTION('',(1.,0.,0.));
#10758=DIRECTION('center_axis',(0.,0.,-1.));
#10759=DIRECTION('ref_axis',(0.,1.,0.));
#10760=DIRECTION('',(0.,1.,0.));
#10761=DIRECTION('',(0.,1.,0.));
#10762=DIRECTION('',(1.,0.,0.));
#10763=DIRECTION('center_axis',(0.,-1.,0.));
#10764=DIRECTION('ref_axis',(0.,0.,-1.));
#10765=DIRECTION('',(0.,0.,-1.));
#10766=DIRECTION('',(0.,0.,-1.));
#10767=DIRECTION('center_axis',(1.,0.,0.));
#10768=DIRECTION('ref_axis',(0.,0.,-1.));
#10769=DIRECTION('center_axis',(1.,0.,0.));
#10770=DIRECTION('ref_axis',(0.,0.,-1.));
#13112=CARTESIAN_POINT('',(0.,0.,0.));
#13113=CARTESIAN_POINT('Origin',(14.,0.,0.97));
#13114=CARTESIAN_POINT('',(13.625,-4.59242549680257E-17,0.97));
#13115=CARTESIAN_POINT('Origin',(14.,0.,0.97));
#13116=CARTESIAN_POINT('',(13.625,4.59242549680257E-17,1.5));
#13117=CARTESIAN_POINT('',(13.625,-4.59242549680257E-17,0.97));
#13118=CARTESIAN_POINT('Origin',(14.,0.,1.5));
#13119=CARTESIAN_POINT('Origin',(14.,0.,0.97));
#13120=CARTESIAN_POINT('',(13.775,-2.75545529808154E-17,0.97));
#13121=CARTESIAN_POINT('Origin',(14.,0.,0.97));
#13122=CARTESIAN_POINT('Origin',(8.,0.,0.97));
#13123=CARTESIAN_POINT('',(7.625,-4.59242549680257E-17,0.97));
#13124=CARTESIAN_POINT('Origin',(8.,0.,0.97));
#13125=CARTESIAN_POINT('',(7.625,4.59242549680257E-17,1.5));
#13126=CARTESIAN_POINT('',(7.625,-4.59242549680257E-17,0.97));
#13127=CARTESIAN_POINT('Origin',(8.,0.,1.5));
#13128=CARTESIAN_POINT('Origin',(8.,0.,0.97));
#13129=CARTESIAN_POINT('',(7.775,-2.75545529808154E-17,0.97));
#13130=CARTESIAN_POINT('Origin',(8.,0.,0.97));
#13131=CARTESIAN_POINT('Origin',(2.,0.,0.97));
#13132=CARTESIAN_POINT('',(1.625,-4.59242549680257E-17,0.97));
#13133=CARTESIAN_POINT('Origin',(2.,0.,0.97));
#13134=CARTESIAN_POINT('',(1.625,4.59242549680257E-17,1.5));
#13135=CARTESIAN_POINT('',(1.625,-4.59242549680257E-17,0.97));
#13136=CARTESIAN_POINT('Origin',(2.,0.,1.5));
#13137=CARTESIAN_POINT('Origin',(2.,0.,0.97));
#13138=CARTESIAN_POINT('',(1.775,-2.75545529808155E-17,0.97));
#13139=CARTESIAN_POINT('Origin',(2.,0.,0.97));
#13140=CARTESIAN_POINT('Origin',(20.,0.,0.97));
#13141=CARTESIAN_POINT('',(19.625,-4.59242549680257E-17,0.97));
#13142=CARTESIAN_POINT('Origin',(20.,0.,0.97));
#13143=CARTESIAN_POINT('',(19.625,4.59242549680257E-17,1.5));
#13144=CARTESIAN_POINT('',(19.625,-4.59242549680257E-17,0.97));
#13145=CARTESIAN_POINT('Origin',(20.,0.,1.5));
#13146=CARTESIAN_POINT('Origin',(20.,0.,0.97));
#13147=CARTESIAN_POINT('',(19.775,-2.75545529808156E-17,0.97));
#13148=CARTESIAN_POINT('Origin',(20.,0.,0.97));
#13149=CARTESIAN_POINT('Origin',(14.,0.,-0.1));
#13150=CARTESIAN_POINT('',(13.775,-2.75545529808154E-17,0.));
#13151=CARTESIAN_POINT('Origin',(14.,0.,0.));
#13152=CARTESIAN_POINT('',(13.775,-2.75545529808154E-17,-0.1));
#13153=CARTESIAN_POINT('Origin',(8.,0.,-0.1));
#13154=CARTESIAN_POINT('',(7.775,-2.75545529808154E-17,0.));
#13155=CARTESIAN_POINT('Origin',(8.,0.,0.));
#13156=CARTESIAN_POINT('',(7.775,-2.75545529808154E-17,-0.1));
#13157=CARTESIAN_POINT('Origin',(2.,0.,-0.1));
#13158=CARTESIAN_POINT('',(1.775,-2.75545529808155E-17,0.));
#13159=CARTESIAN_POINT('Origin',(2.,0.,0.));
#13160=CARTESIAN_POINT('',(1.775,-2.75545529808155E-17,-0.1));
#13161=CARTESIAN_POINT('Origin',(20.,0.,-0.1));
#13162=CARTESIAN_POINT('',(19.775,-2.75545529808156E-17,0.));
#13163=CARTESIAN_POINT('Origin',(20.,0.,0.));
#13164=CARTESIAN_POINT('',(19.775,-2.75545529808156E-17,-0.1));
#13165=CARTESIAN_POINT('Origin',(0.,-0.53,1.));
#13166=CARTESIAN_POINT('',(0.,-0.53,1.));
#13167=CARTESIAN_POINT('',(0.,-0.75,0.85));
#13168=CARTESIAN_POINT('',(0.,-0.53,1.));
#13169=CARTESIAN_POINT('',(22.,-0.75,0.85));
#13170=CARTESIAN_POINT('',(0.,-0.75,0.85));
#13171=CARTESIAN_POINT('',(22.,-0.53,1.));
#13172=CARTESIAN_POINT('',(22.,-0.53,1.));
#13173=CARTESIAN_POINT('',(0.,-0.53,1.));
#13174=CARTESIAN_POINT('Origin',(0.,-0.53,1.15));
#13175=CARTESIAN_POINT('',(0.,-0.53,1.15));
#13176=CARTESIAN_POINT('',(0.,-0.53,1.15));
#13177=CARTESIAN_POINT('',(22.,-0.53,1.15));
#13178=CARTESIAN_POINT('',(22.,-0.53,1.15));
#13179=CARTESIAN_POINT('',(0.,-0.53,1.15));
#13180=CARTESIAN_POINT('Origin',(0.,-0.75,1.3));
#13181=CARTESIAN_POINT('',(0.,-0.75,1.3));
#13182=CARTESIAN_POINT('',(0.,-0.75,1.3));
#13183=CARTESIAN_POINT('',(22.,-0.75,1.3));
#13184=CARTESIAN_POINT('',(22.,-0.75,1.3));
#13185=CARTESIAN_POINT('',(0.,-0.75,1.3));
#13186=CARTESIAN_POINT('Origin',(0.,-0.75,1.5));
#13187=CARTESIAN_POINT('',(0.,-0.75,1.5));
#13188=CARTESIAN_POINT('',(0.,-0.75,1.5));
#13189=CARTESIAN_POINT('',(22.,-0.75,1.5));
#13190=CARTESIAN_POINT('',(22.,-0.75,1.5));
#13191=CARTESIAN_POINT('',(0.,-0.75,1.5));
#13192=CARTESIAN_POINT('Origin',(0.,0.75,1.5));
#13193=CARTESIAN_POINT('',(0.,0.75,1.5));
#13194=CARTESIAN_POINT('',(0.,0.75,1.5));
#13195=CARTESIAN_POINT('',(22.,0.75,1.5));
#13196=CARTESIAN_POINT('',(22.,0.75,1.5));
#13197=CARTESIAN_POINT('',(0.,0.75,1.5));
#13198=CARTESIAN_POINT('Origin',(0.,0.75,1.3));
#13199=CARTESIAN_POINT('',(0.,0.75,1.3));
#13200=CARTESIAN_POINT('',(0.,0.75,1.3));
#13201=CARTESIAN_POINT('',(22.,0.75,1.3));
#13202=CARTESIAN_POINT('',(22.,0.75,1.3));
#13203=CARTESIAN_POINT('',(0.,0.75,1.3));
#13204=CARTESIAN_POINT('Origin',(0.,0.53,1.15));
#13205=CARTESIAN_POINT('',(0.,0.53,1.15));
#13206=CARTESIAN_POINT('',(0.,0.53,1.15));
#13207=CARTESIAN_POINT('',(22.,0.53,1.15));
#13208=CARTESIAN_POINT('',(22.,0.53,1.15));
#13209=CARTESIAN_POINT('',(0.,0.53,1.15));
#13210=CARTESIAN_POINT('Origin',(0.,0.53,1.));
#13211=CARTESIAN_POINT('',(0.,0.53,1.));
#13212=CARTESIAN_POINT('',(0.,0.53,1.));
#13213=CARTESIAN_POINT('',(22.,0.53,1.));
#13214=CARTESIAN_POINT('',(22.,0.53,1.));
#13215=CARTESIAN_POINT('',(0.,0.53,1.));
#13216=CARTESIAN_POINT('Origin',(0.,0.75,0.85));
#13217=CARTESIAN_POINT('',(0.,0.75,0.85));
#13218=CARTESIAN_POINT('',(0.,0.75,0.85));
#13219=CARTESIAN_POINT('',(22.,0.75,0.85));
#13220=CARTESIAN_POINT('',(22.,0.75,0.85));
#13221=CARTESIAN_POINT('',(0.,0.75,0.85));
#13222=CARTESIAN_POINT('Origin',(0.,0.75,0.));
#13223=CARTESIAN_POINT('',(0.,0.75,0.));
#13224=CARTESIAN_POINT('',(0.,0.75,0.));
#13225=CARTESIAN_POINT('',(22.,0.75,0.));
#13226=CARTESIAN_POINT('',(22.,0.75,0.));
#13227=CARTESIAN_POINT('',(0.,0.75,0.));
#13228=CARTESIAN_POINT('Origin',(0.,-0.75,0.));
#13229=CARTESIAN_POINT('',(0.,-0.75,0.));
#13230=CARTESIAN_POINT('',(0.,-0.75,0.));
#13231=CARTESIAN_POINT('',(22.,-0.75,0.));
#13232=CARTESIAN_POINT('',(22.,-0.75,0.));
#13233=CARTESIAN_POINT('',(0.,-0.75,0.));
#13234=CARTESIAN_POINT('Origin',(0.,-0.75,0.85));
#13235=CARTESIAN_POINT('',(0.,-0.75,0.85));
#13236=CARTESIAN_POINT('',(22.,-0.75,0.85));
#13237=CARTESIAN_POINT('Origin',(22.,0.,0.75));
#13238=CARTESIAN_POINT('Origin',(0.,0.,0.75));
#14427=UNCERTAINTY_MEASURE_WITH_UNIT(LENGTH_MEASURE(0.001),#14479,
'DISTANCE_ACCURACY_VALUE',
'Maximum model space distance between geometric entities at asserted c
onnectivities');
#14446=UNCERTAINTY_MEASURE_WITH_UNIT(LENGTH_MEASURE(0.001),#14479,
'DISTANCE_ACCURACY_VALUE',
'Maximum model space distance between geometric entities at asserted c
onnectivities');
#14459=(
GEOMETRIC_REPRESENTATION_CONTEXT(3)
GLOBAL_UNCERTAINTY_ASSIGNED_CONTEXT((#14427))
GLOBAL_UNIT_ASSIGNED_CONTEXT((#14479,#14481,#14482))
REPRESENTATION_CONTEXT('','3D')
);
#14478=(
GEOMETRIC_REPRESENTATION_CONTEXT(3)
GLOBAL_UNCERTAINTY_ASSIGNED_CONTEXT((#14446))
GLOBAL_UNIT_ASSIGNED_CONTEXT((#14479,#14481,#14482))
REPRESENTATION_CONTEXT('','3D')
);
#14479=(
LENGTH_UNIT()
NAMED_UNIT(*)
SI_UNIT(.CENTI.,.METRE.)
);
#14481=(
NAMED_UNIT(*)
PLANE_ANGLE_UNIT()
SI_UNIT($,.RADIAN.)
);
#14482=(
NAMED_UNIT(*)
SI_UNIT($,.STERADIAN.)
SOLID_ANGLE_UNIT()
);
#14495=SHAPE_DEFINITION_REPRESENTATION(#14526,#14615);
#14526=PRODUCT_DEFINITION_SHAPE('',$,#14647);
#14615=SHAPE_REPRESENTATION('',(#9183),#14459);
#14634=PRODUCT_DEFINITION_CONTEXT('part definition',#14729,'design');
#14647=PRODUCT_DEFINITION('Linear Guide Rail - 15 mm, 220 mm Long',
'Linear Guide Rail - 15 mm, 220 mm Long',#14678,#14634);
#14678=PRODUCT_DEFINITION_FORMATION('',$,#14743);
#14729=APPLICATION_CONTEXT(
'Core Data for Automotive Mechanical Design Process');
#14730=PRODUCT_CONTEXT('part definition',#14729,'mechanical');
#14743=PRODUCT('Linear Guide Rail - 15 mm, 220 mm Long',
'Linear Guide Rail - 15 mm, 220 mm Long',
'Linear Guide Rail - 15 mm, 220 mm Long',(#14730));
#14818=COLOUR_RGB('Sky Blue',0.24,0.69,0.87);
#14819=FILL_AREA_STYLE_COLOUR('',#14818);
#14820=FILL_AREA_STYLE('',(#14819));
#14821=SURFACE_STYLE_FILL_AREA(#14820);
#14822=SURFACE_SIDE_STYLE('',(#14821));
#14823=SURFACE_STYLE_USAGE(.BOTH.,#14822);
#14824=PRESENTATION_STYLE_ASSIGNMENT((#14823));
ENDSEC;
END-ISO-10303-21;
